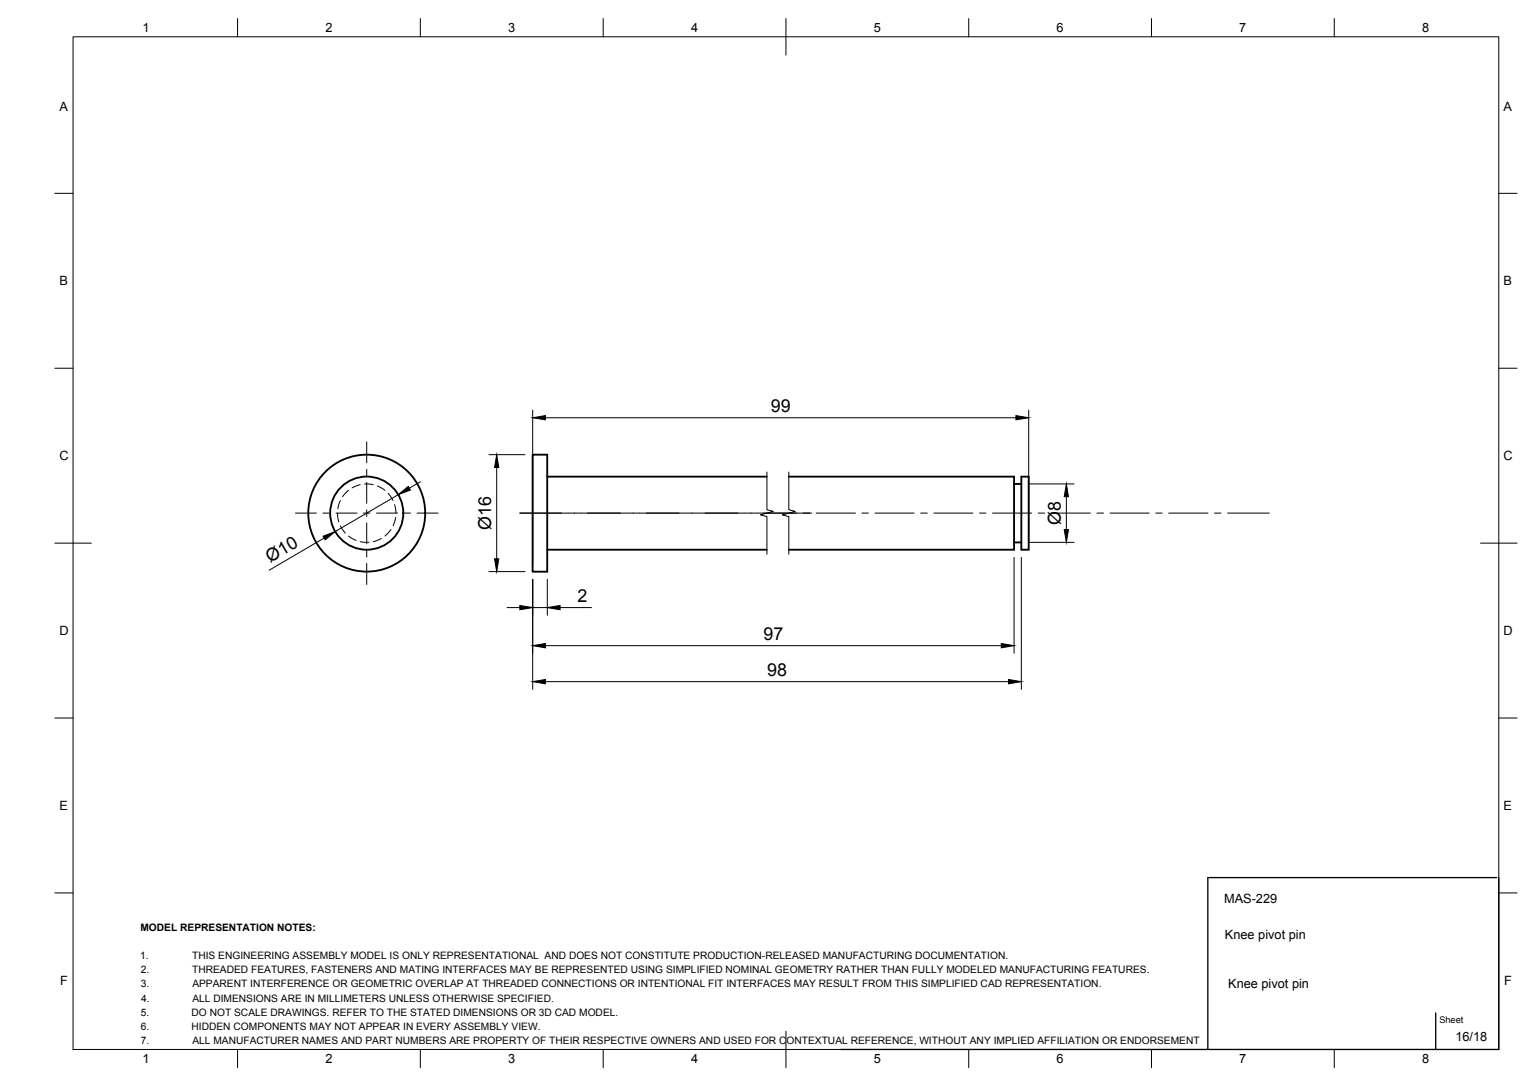
ISO-10303-21;
HEADER;
/* Generated by software containing ST-Developer
 * from STEP Tools, Inc. (www.steptools.com) 
 */

FILE_DESCRIPTION(
/* description */ ('Independently dimensioned six-bar single-leg walking-linkage demonstr
ator. Whole-mm20 crank,60 upper rocker,80/120 ternary coupler,120 lowe
r rocker,140 knee pitch and260 toe reach; ground pivots0/0,60/0,40/60.
 Seven native revolutes close both loops. Four reused native library f
amilies, fully retained shared pins and layered real spacer stacks, bo
nded rubber toe. Benchtop reference mechanism; no complete vehicle, lo
ad, gait stability, adhesive, weld, fit or life rating.'),
/* implementation_level */ '2;1');

FILE_NAME(
/* name */ 'Knee pivot pin.step',
/* time_stamp */ '2026-11-09T20:33:14-08:00',
/* author */ (''),
/* organization */ (''),
/* preprocessor_version */ 'ST-DEVELOPER v20.2',
/* originating_system */ 'Autodesk Translation Framework v15.17.0.0',
/* authorisation */ '');

FILE_SCHEMA (('AUTOMOTIVE_DESIGN { 1 0 10303 214 3 1 1 }'));
ENDSEC;

DATA;
#10=MECHANICAL_DESIGN_GEOMETRIC_PRESENTATION_REPRESENTATION('',(#267),#4048);
#231=SHAPE_REPRESENTATION_RELATIONSHIP('SRR','None',#4155,#249);
#249=ADVANCED_BREP_SHAPE_REPRESENTATION('',(#285),#4042);
#267=STYLED_ITEM('',(#4251),#285);
#285=MANIFOLD_SOLID_BREP('Body1',#2156);
#336=FACE_BOUND('',#678,.T.);
#337=FACE_BOUND('',#680,.T.);
#338=FACE_BOUND('',#683,.T.);
#395=PLANE('',#2550);
#396=PLANE('',#2552);
#397=PLANE('',#2556);
#398=PLANE('',#2561);
#399=PLANE('',#2563);
#505=FACE_OUTER_BOUND('',#676,.T.);
#506=FACE_OUTER_BOUND('',#677,.T.);
#507=FACE_OUTER_BOUND('',#679,.T.);
#508=FACE_OUTER_BOUND('',#681,.T.);
#509=FACE_OUTER_BOUND('',#682,.T.);
#510=FACE_OUTER_BOUND('',#684,.T.);
#511=FACE_OUTER_BOUND('',#685,.T.);
#512=FACE_OUTER_BOUND('',#686,.T.);
#513=FACE_OUTER_BOUND('',#687,.T.);
#676=EDGE_LOOP('',(#1855,#1856,#1857,#1858));
#677=EDGE_LOOP('',(#1859));
#678=EDGE_LOOP('',(#1860));
#679=EDGE_LOOP('',(#1861));
#680=EDGE_LOOP('',(#1862));
#681=EDGE_LOOP('',(#1863,#1864,#1865,#1866));
#682=EDGE_LOOP('',(#1867));
#683=EDGE_LOOP('',(#1868));
#684=EDGE_LOOP('',(#1869,#1870,#1871,#1872));
#685=EDGE_LOOP('',(#1873));
#686=EDGE_LOOP('',(#1874,#1875,#1876,#1877));
#687=EDGE_LOOP('',(#1878));
#827=LINE('',#3831,#952);
#828=LINE('',#3842,#953);
#829=LINE('',#3850,#954);
#830=LINE('',#3854,#955);
#952=VECTOR('',#3150,4.);
#953=VECTOR('',#3165,5.);
#954=VECTOR('',#3174,8.);
#955=VECTOR('',#3181,5.);
#1056=CIRCLE('',#2548,4.);
#1057=CIRCLE('',#2549,4.);
#1058=CIRCLE('',#2551,5.);
#1059=CIRCLE('',#2553,5.);
#1060=CIRCLE('',#2555,5.);
#1061=CIRCLE('',#2557,8.);
#1062=CIRCLE('',#2558,5.);
#1063=CIRCLE('',#2560,8.);
#1210=VERTEX_POINT('',#3828);
#1211=VERTEX_POINT('',#3830);
#1212=VERTEX_POINT('',#3834);
#1213=VERTEX_POINT('',#3837);
#1214=VERTEX_POINT('',#3840);
#1215=VERTEX_POINT('',#3844);
#1216=VERTEX_POINT('',#3846);
#1217=VERTEX_POINT('',#3849);
#1431=EDGE_CURVE('',#1210,#1210,#1056,.T.);
#1432=EDGE_CURVE('',#1210,#1211,#827,.T.);
#1433=EDGE_CURVE('',#1211,#1211,#1057,.T.);
#1434=EDGE_CURVE('',#1212,#1212,#1058,.T.);
#1435=EDGE_CURVE('',#1213,#1213,#1059,.T.);
#1436=EDGE_CURVE('',#1214,#1214,#1060,.T.);
#1437=EDGE_CURVE('',#1214,#1213,#828,.T.);
#1438=EDGE_CURVE('',#1215,#1215,#1061,.T.);
#1439=EDGE_CURVE('',#1216,#1216,#1062,.T.);
#1440=EDGE_CURVE('',#1215,#1217,#829,.T.);
#1441=EDGE_CURVE('',#1217,#1217,#1063,.T.);
#1442=EDGE_CURVE('',#1212,#1216,#830,.T.);
#1855=ORIENTED_EDGE('',*,*,#1431,.T.);
#1856=ORIENTED_EDGE('',*,*,#1432,.T.);
#1857=ORIENTED_EDGE('',*,*,#1433,.F.);
#1858=ORIENTED_EDGE('',*,*,#1432,.F.);
#1859=ORIENTED_EDGE('',*,*,#1434,.F.);
#1860=ORIENTED_EDGE('',*,*,#1431,.F.);
#1861=ORIENTED_EDGE('',*,*,#1435,.F.);
#1862=ORIENTED_EDGE('',*,*,#1433,.T.);
#1863=ORIENTED_EDGE('',*,*,#1436,.F.);
#1864=ORIENTED_EDGE('',*,*,#1437,.T.);
#1865=ORIENTED_EDGE('',*,*,#1435,.T.);
#1866=ORIENTED_EDGE('',*,*,#1437,.F.);
#1867=ORIENTED_EDGE('',*,*,#1438,.T.);
#1868=ORIENTED_EDGE('',*,*,#1439,.F.);
#1869=ORIENTED_EDGE('',*,*,#1438,.F.);
#1870=ORIENTED_EDGE('',*,*,#1440,.T.);
#1871=ORIENTED_EDGE('',*,*,#1441,.T.);
#1872=ORIENTED_EDGE('',*,*,#1440,.F.);
#1873=ORIENTED_EDGE('',*,*,#1441,.F.);
#1874=ORIENTED_EDGE('',*,*,#1434,.T.);
#1875=ORIENTED_EDGE('',*,*,#1442,.T.);
#1876=ORIENTED_EDGE('',*,*,#1439,.T.);
#1877=ORIENTED_EDGE('',*,*,#1442,.F.);
#1878=ORIENTED_EDGE('',*,*,#1436,.T.);
#2002=CYLINDRICAL_SURFACE('',#2547,4.);
#2003=CYLINDRICAL_SURFACE('',#2554,5.);
#2004=CYLINDRICAL_SURFACE('',#2559,8.);
#2005=CYLINDRICAL_SURFACE('',#2562,5.);
#2108=ADVANCED_FACE('',(#505),#2002,.T.);
#2109=ADVANCED_FACE('',(#506,#336),#395,.F.);
#2110=ADVANCED_FACE('',(#507,#337),#396,.F.);
#2111=ADVANCED_FACE('',(#508),#2003,.T.);
#2112=ADVANCED_FACE('',(#509,#338),#397,.T.);
#2113=ADVANCED_FACE('',(#510),#2004,.T.);
#2114=ADVANCED_FACE('',(#511),#398,.F.);
#2115=ADVANCED_FACE('',(#512),#2005,.T.);
#2116=ADVANCED_FACE('',(#513),#399,.T.);
#2156=CLOSED_SHELL('',(#2108,#2109,#2110,#2111,#2112,#2113,#2114,#2115,
#2116));
#2546=AXIS2_PLACEMENT_3D('',#3826,#3144,#3145);
#2547=AXIS2_PLACEMENT_3D('',#3827,#3146,#3147);
#2548=AXIS2_PLACEMENT_3D('',#3829,#3148,#3149);
#2549=AXIS2_PLACEMENT_3D('',#3832,#3151,#3152);
#2550=AXIS2_PLACEMENT_3D('',#3833,#3153,#3154);
#2551=AXIS2_PLACEMENT_3D('',#3835,#3155,#3156);
#2552=AXIS2_PLACEMENT_3D('',#3836,#3157,#3158);
#2553=AXIS2_PLACEMENT_3D('',#3838,#3159,#3160);
#2554=AXIS2_PLACEMENT_3D('',#3839,#3161,#3162);
#2555=AXIS2_PLACEMENT_3D('',#3841,#3163,#3164);
#2556=AXIS2_PLACEMENT_3D('',#3843,#3166,#3167);
#2557=AXIS2_PLACEMENT_3D('',#3845,#3168,#3169);
#2558=AXIS2_PLACEMENT_3D('',#3847,#3170,#3171);
#2559=AXIS2_PLACEMENT_3D('',#3848,#3172,#3173);
#2560=AXIS2_PLACEMENT_3D('',#3851,#3175,#3176);
#2561=AXIS2_PLACEMENT_3D('',#3852,#3177,#3178);
#2562=AXIS2_PLACEMENT_3D('',#3853,#3179,#3180);
#2563=AXIS2_PLACEMENT_3D('',#3855,#3182,#3183);
#3144=DIRECTION('axis',(0.,0.,1.));
#3145=DIRECTION('refdir',(1.,0.,0.));
#3146=DIRECTION('center_axis',(0.,0.,1.));
#3147=DIRECTION('ref_axis',(1.,0.,0.));
#3148=DIRECTION('center_axis',(0.,0.,1.));
#3149=DIRECTION('ref_axis',(1.,0.,0.));
#3150=DIRECTION('',(0.,0.,1.));
#3151=DIRECTION('center_axis',(0.,0.,1.));
#3152=DIRECTION('ref_axis',(1.,0.,0.));
#3153=DIRECTION('center_axis',(0.,0.,-1.));
#3154=DIRECTION('ref_axis',(-1.,0.,0.));
#3155=DIRECTION('center_axis',(0.,0.,-1.));
#3156=DIRECTION('ref_axis',(1.,0.,0.));
#3157=DIRECTION('center_axis',(0.,0.,1.));
#3158=DIRECTION('ref_axis',(1.,0.,0.));
#3159=DIRECTION('center_axis',(0.,0.,1.));
#3160=DIRECTION('ref_axis',(1.,0.,0.));
#3161=DIRECTION('center_axis',(0.,0.,1.));
#3162=DIRECTION('ref_axis',(1.,0.,0.));
#3163=DIRECTION('center_axis',(0.,0.,1.));
#3164=DIRECTION('ref_axis',(1.,0.,0.));
#3165=DIRECTION('',(0.,0.,-1.));
#3166=DIRECTION('center_axis',(0.,0.,1.));
#3167=DIRECTION('ref_axis',(1.,0.,0.));
#3168=DIRECTION('center_axis',(0.,0.,1.));
#3169=DIRECTION('ref_axis',(1.,0.,0.));
#3170=DIRECTION('center_axis',(0.,0.,1.));
#3171=DIRECTION('ref_axis',(1.,0.,0.));
#3172=DIRECTION('center_axis',(0.,0.,1.));
#3173=DIRECTION('ref_axis',(1.,0.,0.));
#3174=DIRECTION('',(0.,0.,-1.));
#3175=DIRECTION('center_axis',(0.,0.,1.));
#3176=DIRECTION('ref_axis',(1.,0.,0.));
#3177=DIRECTION('center_axis',(0.,0.,1.));
#3178=DIRECTION('ref_axis',(1.,0.,0.));
#3179=DIRECTION('center_axis',(0.,0.,1.));
#3180=DIRECTION('ref_axis',(1.,0.,0.));
#3181=DIRECTION('',(0.,0.,-1.));
#3182=DIRECTION('center_axis',(0.,0.,1.));
#3183=DIRECTION('ref_axis',(1.,0.,0.));
#3826=CARTESIAN_POINT('',(0.,0.,0.));
#3827=CARTESIAN_POINT('Origin',(0.,0.,95.5));
#3828=CARTESIAN_POINT('',(-4.,-4.89858719658941E-16,95.));
#3829=CARTESIAN_POINT('Origin',(0.,0.,95.));
#3830=CARTESIAN_POINT('',(-4.,-4.89858719658941E-16,96.));
#3831=CARTESIAN_POINT('',(-4.,-4.89858719658941E-16,95.5));
#3832=CARTESIAN_POINT('Origin',(0.,0.,96.));
#3833=CARTESIAN_POINT('Origin',(8.,0.,95.));
#3834=CARTESIAN_POINT('',(-5.,6.12323399573677E-16,95.));
#3835=CARTESIAN_POINT('Origin',(0.,0.,95.));
#3836=CARTESIAN_POINT('Origin',(4.,0.,96.));
#3837=CARTESIAN_POINT('',(-5.,-6.12323399573677E-16,96.));
#3838=CARTESIAN_POINT('Origin',(0.,0.,96.));
#3839=CARTESIAN_POINT('Origin',(0.,0.,0.));
#3840=CARTESIAN_POINT('',(-5.,-6.12323399573677E-16,97.));
#3841=CARTESIAN_POINT('Origin',(0.,0.,97.));
#3842=CARTESIAN_POINT('',(-5.,-6.12323399573677E-16,0.));
#3843=CARTESIAN_POINT('Origin',(0.,0.,0.));
#3844=CARTESIAN_POINT('',(-8.,-9.79717439317883E-16,0.));
#3845=CARTESIAN_POINT('Origin',(0.,0.,0.));
#3846=CARTESIAN_POINT('',(-5.,-6.12323399573677E-16,0.));
#3847=CARTESIAN_POINT('Origin',(0.,0.,0.));
#3848=CARTESIAN_POINT('Origin',(0.,0.,-2.));
#3849=CARTESIAN_POINT('',(-8.,-9.79717439317883E-16,-2.));
#3850=CARTESIAN_POINT('',(-8.,-9.79717439317883E-16,-2.));
#3851=CARTESIAN_POINT('Origin',(0.,0.,-2.));
#3852=CARTESIAN_POINT('Origin',(0.,0.,-2.));
#3853=CARTESIAN_POINT('Origin',(0.,0.,0.));
#3854=CARTESIAN_POINT('',(-5.,-6.12323399573677E-16,0.));
#3855=CARTESIAN_POINT('Origin',(0.,0.,97.));
#4022=UNCERTAINTY_MEASURE_WITH_UNIT(LENGTH_MEASURE(0.01),#4049,
'DISTANCE_ACCURACY_VALUE',
'Maximum model space distance between geometric entities at asserted c
onnectivities');
#4028=UNCERTAINTY_MEASURE_WITH_UNIT(LENGTH_MEASURE(0.01),#4049,
'DISTANCE_ACCURACY_VALUE',
'Maximum model space distance between geometric entities at asserted c
onnectivities');
#4042=(
GEOMETRIC_REPRESENTATION_CONTEXT(3)
GLOBAL_UNCERTAINTY_ASSIGNED_CONTEXT((#4022))
GLOBAL_UNIT_ASSIGNED_CONTEXT((#4049,#4051,#4052))
REPRESENTATION_CONTEXT('','3D')
);
#4048=(
GEOMETRIC_REPRESENTATION_CONTEXT(3)
GLOBAL_UNCERTAINTY_ASSIGNED_CONTEXT((#4028))
GLOBAL_UNIT_ASSIGNED_CONTEXT((#4049,#4051,#4052))
REPRESENTATION_CONTEXT('','3D')
);
#4049=(
LENGTH_UNIT()
NAMED_UNIT(*)
SI_UNIT(.MILLI.,.METRE.)
);
#4051=(
NAMED_UNIT(*)
PLANE_ANGLE_UNIT()
SI_UNIT($,.RADIAN.)
);
#4052=(
NAMED_UNIT(*)
SI_UNIT($,.STERADIAN.)
SOLID_ANGLE_UNIT()
);
#4066=SHAPE_DEFINITION_REPRESENTATION(#4085,#4155);
#4085=PRODUCT_DEFINITION_SHAPE('',$,#4175);
#4155=SHAPE_REPRESENTATION('',(#2546),#4042);
#4161=PRODUCT_DEFINITION_CONTEXT('part definition',#4220,'design');
#4175=PRODUCT_DEFINITION('Knee pivot pin','Knee pivot pin',#4194,#4161);
#4194=PRODUCT_DEFINITION_FORMATION('',$,#4235);
#4220=APPLICATION_CONTEXT(
'Core Data for Automotive Mechanical Design Process');
#4221=PRODUCT_CONTEXT('part definition',#4220,'mechanical');
#4235=PRODUCT('Knee pivot pin','Knee pivot pin',$,(#4221));
#4251=PRESENTATION_STYLE_ASSIGNMENT((#4265));
#4265=SURFACE_STYLE_USAGE(.BOTH.,#4279);
#4279=SURFACE_SIDE_STYLE('',(#4293));
#4293=SURFACE_STYLE_FILL_AREA(#4307);
#4307=FILL_AREA_STYLE('Pin gray',(#4321));
#4321=FILL_AREA_STYLE_COLOUR('Pin gray',#4335);
#4335=COLOUR_RGB('Pin gray',0.576470588235294,0.615686274509804,0.666666666666667);
ENDSEC;
END-ISO-10303-21;
